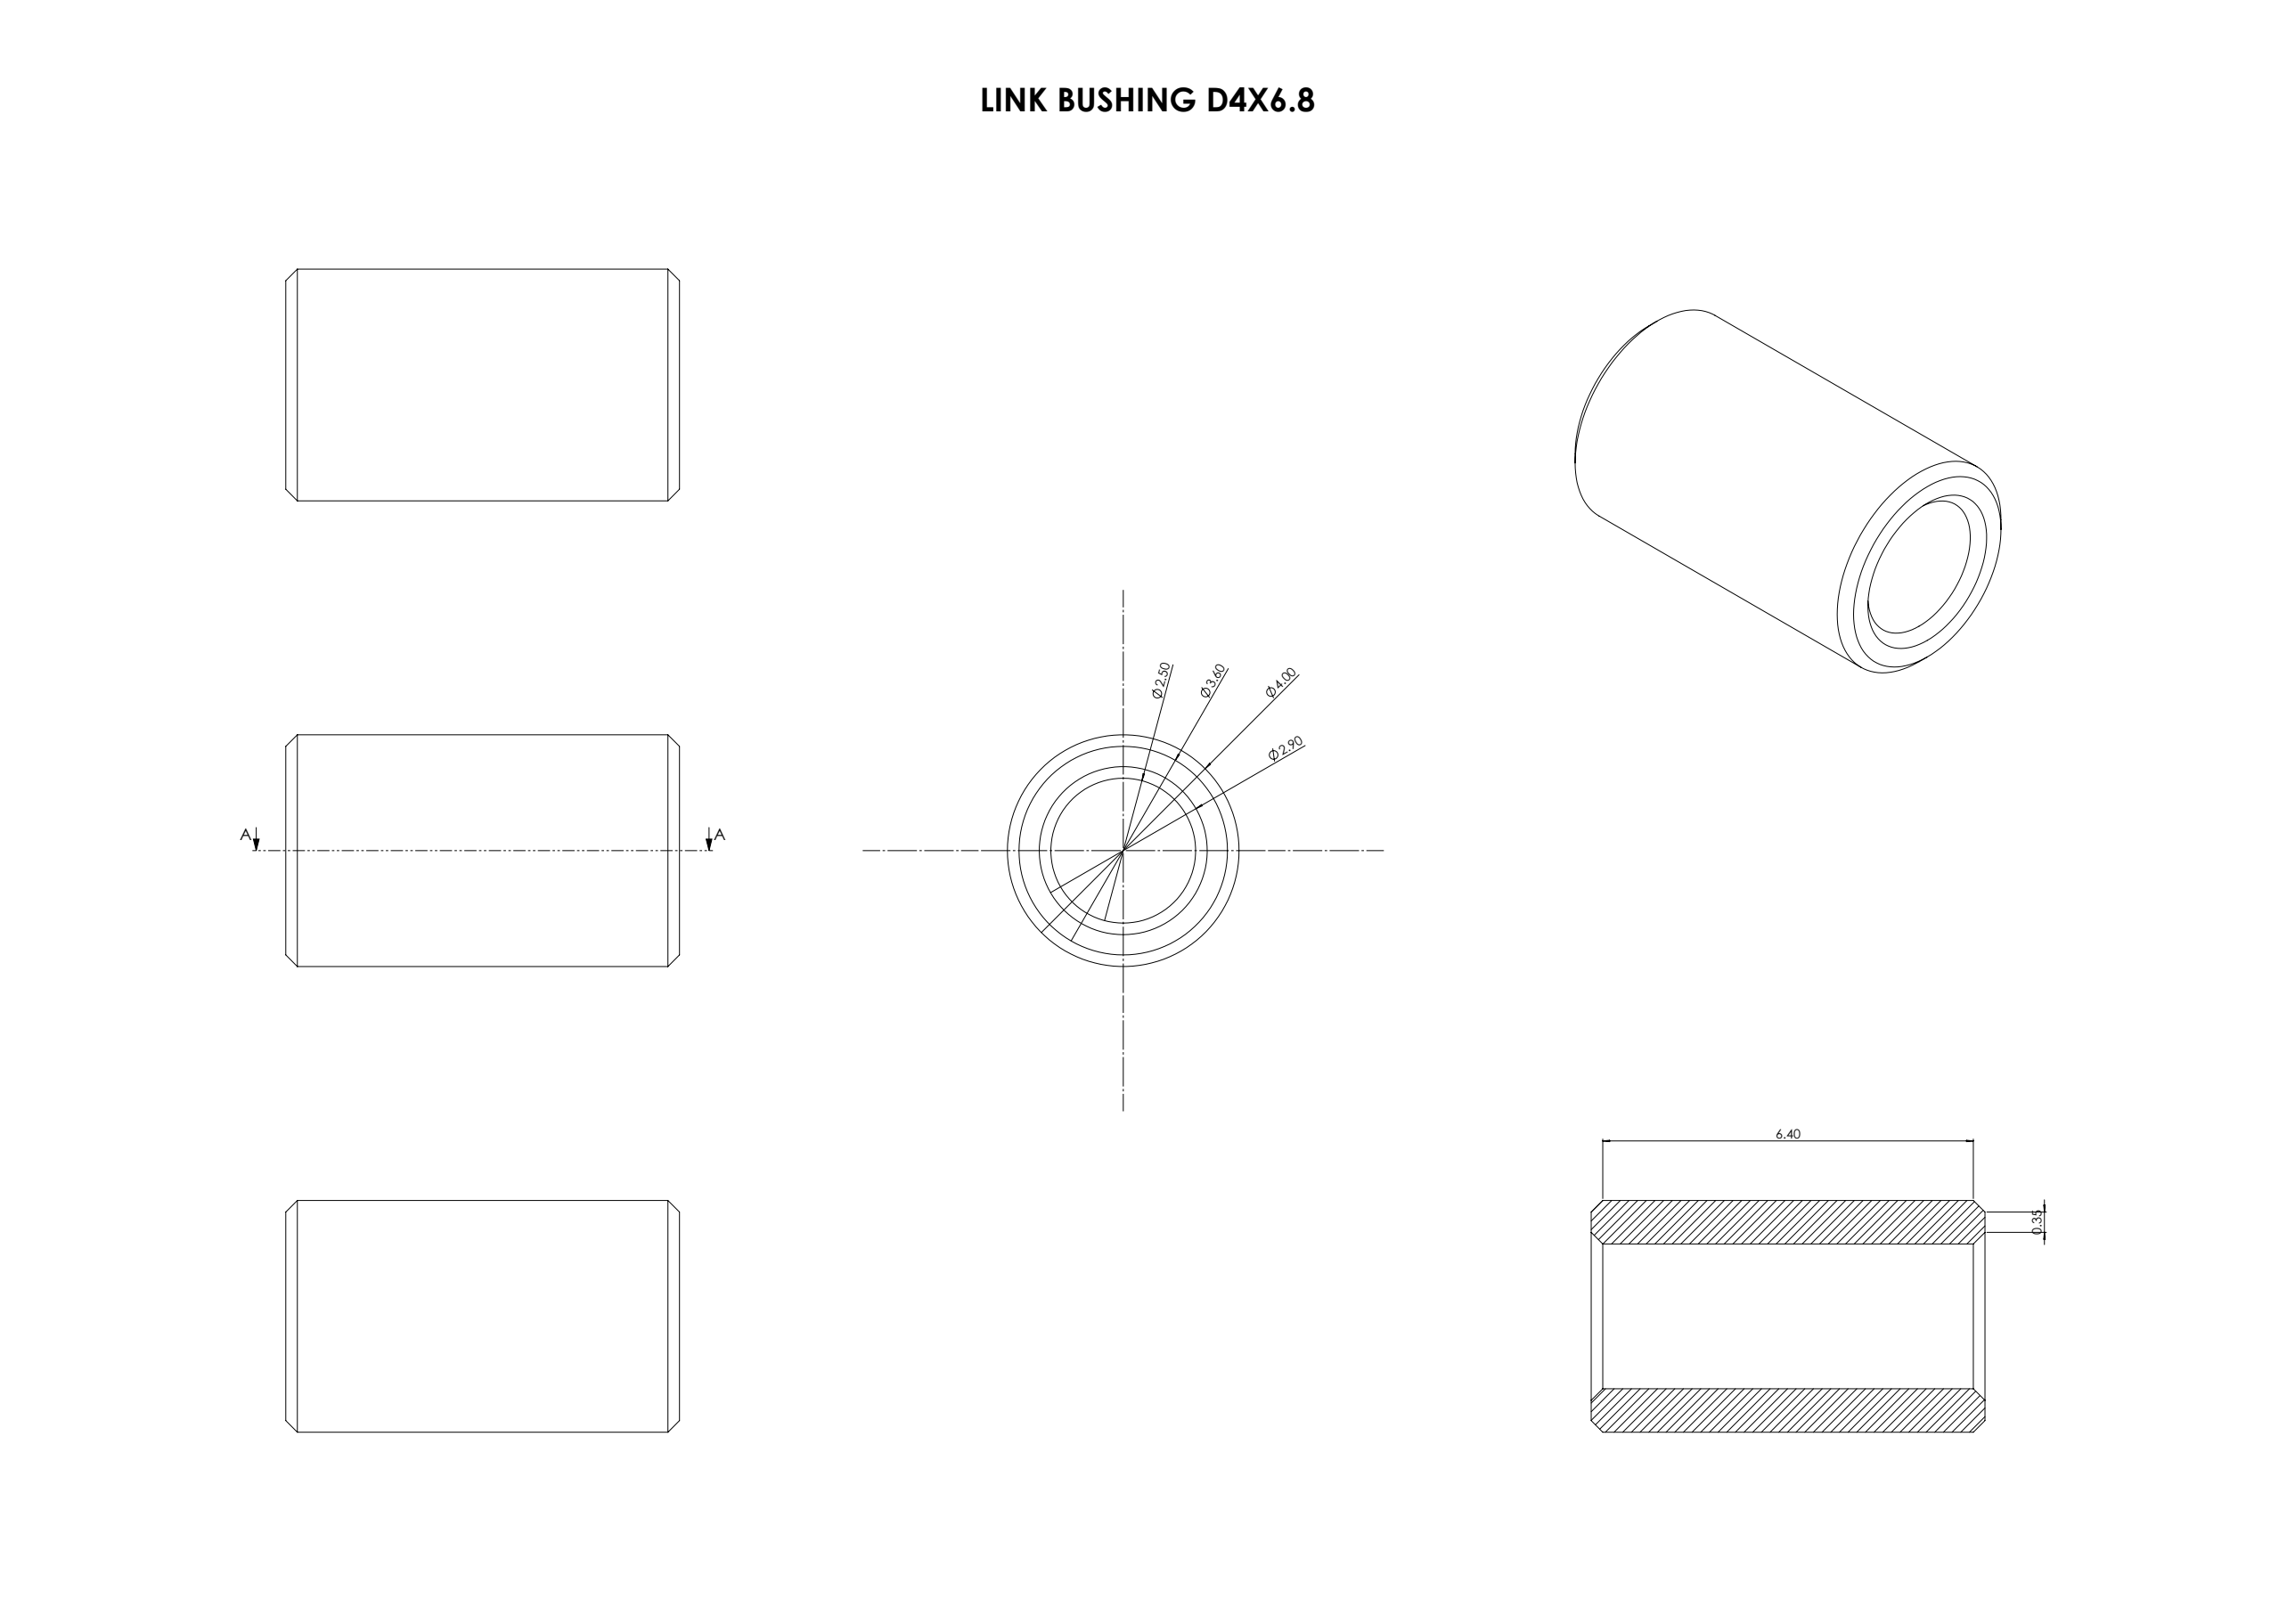
ISO-10303-21;
HEADER;
/* Generated by software containing ST-Developer
 * from STEP Tools, Inc. (www.steptools.com) 
 */

FILE_DESCRIPTION(
/* description */ (''),
/* implementation_level */ '2;1');

FILE_NAME(
/* name */ '10_Link_Bushing_D4x6.8.step',
/* time_stamp */ '2026-10-25T01:35:35-07:00',
/* author */ (''),
/* organization */ (''),
/* preprocessor_version */ 'ST-DEVELOPER v20.2',
/* originating_system */ 'Autodesk Translation Framework v15.15.0.0',
/* authorisation */ '');

FILE_SCHEMA (('AUTOMOTIVE_DESIGN { 1 0 10303 214 3 1 1 }'));
ENDSEC;

DATA;
#10=MECHANICAL_DESIGN_GEOMETRIC_PRESENTATION_REPRESENTATION('',(#271),#11430);
#247=SHAPE_REPRESENTATION_RELATIONSHIP('SRR','None',#11490,#259);
#259=ADVANCED_BREP_SHAPE_REPRESENTATION('',(#283),#11429);
#271=STYLED_ITEM('',(#11623),#283);
#283=MANIFOLD_SOLID_BREP('Body1',#4472);
#321=FACE_BOUND('',#1094,.T.);
#322=FACE_BOUND('',#1097,.T.);
#429=PLANE('',#5055);
#430=PLANE('',#5059);
#524=CYLINDRICAL_SURFACE('',#5052,1.25);
#525=CYLINDRICAL_SURFACE('',#5063,2.);
#786=FACE_OUTER_BOUND('',#1091,.T.);
#787=FACE_OUTER_BOUND('',#1092,.T.);
#788=FACE_OUTER_BOUND('',#1093,.T.);
#789=FACE_OUTER_BOUND('',#1095,.T.);
#790=FACE_OUTER_BOUND('',#1096,.T.);
#791=FACE_OUTER_BOUND('',#1098,.T.);
#792=FACE_OUTER_BOUND('',#1099,.T.);
#793=FACE_OUTER_BOUND('',#1100,.T.);
#1091=EDGE_LOOP('',(#4103,#4104,#4105,#4106,#4107));
#1092=EDGE_LOOP('',(#4108,#4109,#4110,#4111,#4112,#4113));
#1093=EDGE_LOOP('',(#4114));
#1094=EDGE_LOOP('',(#4115));
#1095=EDGE_LOOP('',(#4116,#4117,#4118,#4119,#4120));
#1096=EDGE_LOOP('',(#4121));
#1097=EDGE_LOOP('',(#4122));
#1098=EDGE_LOOP('',(#4123,#4124,#4125,#4126));
#1099=EDGE_LOOP('',(#4127,#4128,#4129,#4130));
#1100=EDGE_LOOP('',(#4131,#4132,#4133,#4134));
#1385=LINE('',#11356,#1675);
#1386=LINE('',#11365,#1676);
#1387=LINE('',#11371,#1677);
#1388=LINE('',#11379,#1678);
#1389=LINE('',#11383,#1679);
#1390=LINE('',#11385,#1680);
#1675=VECTOR('',#6255,1.35);
#1676=VECTOR('',#6266,1.25);
#1677=VECTOR('',#6273,1.35);
#1678=VECTOR('',#6284,1.9);
#1679=VECTOR('',#6289,2.);
#1680=VECTOR('',#6292,1.9);
#1856=CIRCLE('',#5049,1.45);
#1857=CIRCLE('',#5050,1.25);
#1858=CIRCLE('',#5051,1.25);
#1859=CIRCLE('',#5053,1.25);
#1860=CIRCLE('',#5054,1.25);
#1861=CIRCLE('',#5056,1.8);
#1862=CIRCLE('',#5058,1.45);
#1863=CIRCLE('',#5060,1.8);
#1864=CIRCLE('',#5062,2.);
#1865=CIRCLE('',#5064,2.);
#2250=VERTEX_POINT('',#11353);
#2251=VERTEX_POINT('',#11355);
#2252=VERTEX_POINT('',#11357);
#2253=VERTEX_POINT('',#11361);
#2254=VERTEX_POINT('',#11362);
#2255=VERTEX_POINT('',#11367);
#2256=VERTEX_POINT('',#11370);
#2257=VERTEX_POINT('',#11374);
#2258=VERTEX_POINT('',#11377);
#2259=VERTEX_POINT('',#11381);
#2869=EDGE_CURVE('',#2250,#2250,#1856,.T.);
#2870=EDGE_CURVE('',#2250,#2251,#1385,.T.);
#2871=EDGE_CURVE('',#2251,#2252,#1857,.T.);
#2872=EDGE_CURVE('',#2252,#2251,#1858,.T.);
#2873=EDGE_CURVE('',#2253,#2254,#1859,.T.);
#2874=EDGE_CURVE('',#2254,#2253,#1860,.T.);
#2875=EDGE_CURVE('',#2254,#2252,#1386,.T.);
#2876=EDGE_CURVE('',#2255,#2255,#1861,.T.);
#2877=EDGE_CURVE('',#2253,#2256,#1387,.T.);
#2878=EDGE_CURVE('',#2256,#2256,#1862,.T.);
#2879=EDGE_CURVE('',#2257,#2257,#1863,.T.);
#2880=EDGE_CURVE('',#2258,#2258,#1864,.T.);
#2881=EDGE_CURVE('',#2258,#2255,#1388,.T.);
#2882=EDGE_CURVE('',#2259,#2259,#1865,.T.);
#2883=EDGE_CURVE('',#2259,#2258,#1389,.T.);
#2884=EDGE_CURVE('',#2257,#2259,#1390,.T.);
#4103=ORIENTED_EDGE('',*,*,#2869,.T.);
#4104=ORIENTED_EDGE('',*,*,#2870,.T.);
#4105=ORIENTED_EDGE('',*,*,#2871,.T.);
#4106=ORIENTED_EDGE('',*,*,#2872,.T.);
#4107=ORIENTED_EDGE('',*,*,#2870,.F.);
#4108=ORIENTED_EDGE('',*,*,#2873,.F.);
#4109=ORIENTED_EDGE('',*,*,#2874,.F.);
#4110=ORIENTED_EDGE('',*,*,#2875,.T.);
#4111=ORIENTED_EDGE('',*,*,#2871,.F.);
#4112=ORIENTED_EDGE('',*,*,#2872,.F.);
#4113=ORIENTED_EDGE('',*,*,#2875,.F.);
#4114=ORIENTED_EDGE('',*,*,#2876,.F.);
#4115=ORIENTED_EDGE('',*,*,#2869,.F.);
#4116=ORIENTED_EDGE('',*,*,#2873,.T.);
#4117=ORIENTED_EDGE('',*,*,#2874,.T.);
#4118=ORIENTED_EDGE('',*,*,#2877,.T.);
#4119=ORIENTED_EDGE('',*,*,#2878,.T.);
#4120=ORIENTED_EDGE('',*,*,#2877,.F.);
#4121=ORIENTED_EDGE('',*,*,#2879,.T.);
#4122=ORIENTED_EDGE('',*,*,#2878,.F.);
#4123=ORIENTED_EDGE('',*,*,#2880,.F.);
#4124=ORIENTED_EDGE('',*,*,#2881,.T.);
#4125=ORIENTED_EDGE('',*,*,#2876,.T.);
#4126=ORIENTED_EDGE('',*,*,#2881,.F.);
#4127=ORIENTED_EDGE('',*,*,#2882,.F.);
#4128=ORIENTED_EDGE('',*,*,#2883,.T.);
#4129=ORIENTED_EDGE('',*,*,#2880,.T.);
#4130=ORIENTED_EDGE('',*,*,#2883,.F.);
#4131=ORIENTED_EDGE('',*,*,#2879,.F.);
#4132=ORIENTED_EDGE('',*,*,#2884,.T.);
#4133=ORIENTED_EDGE('',*,*,#2882,.T.);
#4134=ORIENTED_EDGE('',*,*,#2884,.F.);
#4189=CONICAL_SURFACE('',#5048,1.35,0.785398163397448);
#4190=CONICAL_SURFACE('',#5057,1.35,0.785398163397448);
#4191=CONICAL_SURFACE('',#5061,1.9,0.785398163397449);
#4192=CONICAL_SURFACE('',#5065,1.9,0.785398163397448);
#4453=ADVANCED_FACE('',(#786),#4189,.F.);
#4454=ADVANCED_FACE('',(#787),#524,.F.);
#4455=ADVANCED_FACE('',(#788,#321),#429,.T.);
#4456=ADVANCED_FACE('',(#789),#4190,.F.);
#4457=ADVANCED_FACE('',(#790,#322),#430,.T.);
#4458=ADVANCED_FACE('',(#791),#4191,.T.);
#4459=ADVANCED_FACE('',(#792),#525,.T.);
#4460=ADVANCED_FACE('',(#793),#4192,.T.);
#4472=CLOSED_SHELL('',(#4453,#4454,#4455,#4456,#4457,#4458,#4459,#4460));
#5047=AXIS2_PLACEMENT_3D('',#11351,#6249,#6250);
#5048=AXIS2_PLACEMENT_3D('',#11352,#6251,#6252);
#5049=AXIS2_PLACEMENT_3D('',#11354,#6253,#6254);
#5050=AXIS2_PLACEMENT_3D('',#11358,#6256,#6257);
#5051=AXIS2_PLACEMENT_3D('',#11359,#6258,#6259);
#5052=AXIS2_PLACEMENT_3D('',#11360,#6260,#6261);
#5053=AXIS2_PLACEMENT_3D('',#11363,#6262,#6263);
#5054=AXIS2_PLACEMENT_3D('',#11364,#6264,#6265);
#5055=AXIS2_PLACEMENT_3D('',#11366,#6267,#6268);
#5056=AXIS2_PLACEMENT_3D('',#11368,#6269,#6270);
#5057=AXIS2_PLACEMENT_3D('',#11369,#6271,#6272);
#5058=AXIS2_PLACEMENT_3D('',#11372,#6274,#6275);
#5059=AXIS2_PLACEMENT_3D('',#11373,#6276,#6277);
#5060=AXIS2_PLACEMENT_3D('',#11375,#6278,#6279);
#5061=AXIS2_PLACEMENT_3D('',#11376,#6280,#6281);
#5062=AXIS2_PLACEMENT_3D('',#11378,#6282,#6283);
#5063=AXIS2_PLACEMENT_3D('',#11380,#6285,#6286);
#5064=AXIS2_PLACEMENT_3D('',#11382,#6287,#6288);
#5065=AXIS2_PLACEMENT_3D('',#11384,#6290,#6291);
#6249=DIRECTION('axis',(0.,0.,1.));
#6250=DIRECTION('refdir',(1.,0.,0.));
#6251=DIRECTION('center_axis',(-1.,0.,0.));
#6252=DIRECTION('ref_axis',(0.,-1.,0.));
#6253=DIRECTION('center_axis',(-1.,0.,0.));
#6254=DIRECTION('ref_axis',(0.,-1.,0.));
#6255=DIRECTION('',(0.707106781186548,-0.707106781186548,8.65956056235493E-17));
#6256=DIRECTION('center_axis',(1.,0.,0.));
#6257=DIRECTION('ref_axis',(0.,-1.,0.));
#6258=DIRECTION('center_axis',(1.,0.,0.));
#6259=DIRECTION('ref_axis',(0.,-1.,0.));
#6260=DIRECTION('center_axis',(1.,0.,0.));
#6261=DIRECTION('ref_axis',(0.,1.,0.));
#6262=DIRECTION('center_axis',(-1.,0.,0.));
#6263=DIRECTION('ref_axis',(0.,-1.,0.));
#6264=DIRECTION('center_axis',(-1.,0.,0.));
#6265=DIRECTION('ref_axis',(0.,-1.,0.));
#6266=DIRECTION('',(-1.,0.,0.));
#6267=DIRECTION('center_axis',(-1.,0.,0.));
#6268=DIRECTION('ref_axis',(0.,0.,1.));
#6269=DIRECTION('center_axis',(1.,0.,0.));
#6270=DIRECTION('ref_axis',(0.,0.,-1.));
#6271=DIRECTION('center_axis',(1.,0.,0.));
#6272=DIRECTION('ref_axis',(0.,-1.,0.));
#6273=DIRECTION('',(0.707106781186548,0.707106781186548,-8.65956056235493E-17));
#6274=DIRECTION('center_axis',(1.,0.,0.));
#6275=DIRECTION('ref_axis',(0.,-1.,0.));
#6276=DIRECTION('center_axis',(1.,0.,0.));
#6277=DIRECTION('ref_axis',(0.,0.,-1.));
#6278=DIRECTION('center_axis',(1.,0.,0.));
#6279=DIRECTION('ref_axis',(0.,0.,-1.));
#6280=DIRECTION('center_axis',(1.,0.,0.));
#6281=DIRECTION('ref_axis',(0.,1.,0.));
#6282=DIRECTION('center_axis',(1.,0.,0.));
#6283=DIRECTION('ref_axis',(0.,0.,-1.));
#6284=DIRECTION('',(-0.707106781186547,0.707106781186548,8.65956056235494E-17));
#6285=DIRECTION('center_axis',(1.,0.,0.));
#6286=DIRECTION('ref_axis',(0.,1.,0.));
#6287=DIRECTION('center_axis',(1.,0.,0.));
#6288=DIRECTION('ref_axis',(0.,0.,-1.));
#6289=DIRECTION('',(-1.,0.,0.));
#6290=DIRECTION('center_axis',(-1.,0.,0.));
#6291=DIRECTION('ref_axis',(0.,1.,0.));
#6292=DIRECTION('',(-0.707106781186547,-0.707106781186547,-8.65956056235493E-17));
#11351=CARTESIAN_POINT('',(0.,0.,0.));
#11352=CARTESIAN_POINT('Origin',(0.1,0.,0.));
#11353=CARTESIAN_POINT('',(0.,1.45,-1.77573785876366E-16));
#11354=CARTESIAN_POINT('Origin',(0.,0.,0.));
#11355=CARTESIAN_POINT('',(0.2,1.25,1.53080849893419E-16));
#11356=CARTESIAN_POINT('',(0.1,1.35,-1.65327317884893E-16));
#11357=CARTESIAN_POINT('',(0.2,-1.25,-1.53080849893419E-16));
#11358=CARTESIAN_POINT('Origin',(0.2,0.,0.));
#11359=CARTESIAN_POINT('Origin',(0.2,0.,0.));
#11360=CARTESIAN_POINT('Origin',(3.4,0.,0.));
#11361=CARTESIAN_POINT('',(6.6,1.25,-1.53080849893419E-16));
#11362=CARTESIAN_POINT('',(6.6,-1.25,-1.53080849893419E-16));
#11363=CARTESIAN_POINT('Origin',(6.6,0.,0.));
#11364=CARTESIAN_POINT('Origin',(6.6,0.,0.));
#11365=CARTESIAN_POINT('',(3.4,-1.25,-1.53080849893419E-16));
#11366=CARTESIAN_POINT('Origin',(0.,1.8,0.));
#11367=CARTESIAN_POINT('',(1.73472347597681E-17,-1.8,-2.20436423846524E-16));
#11368=CARTESIAN_POINT('Origin',(0.,0.,0.));
#11369=CARTESIAN_POINT('Origin',(6.7,0.,0.));
#11370=CARTESIAN_POINT('',(6.8,1.45,1.77573785876366E-16));
#11371=CARTESIAN_POINT('',(6.7,1.35,-1.65327317884893E-16));
#11372=CARTESIAN_POINT('Origin',(6.8,0.,0.));
#11373=CARTESIAN_POINT('Origin',(6.8,1.25,0.));
#11374=CARTESIAN_POINT('',(6.8,-1.8,-2.20436423846524E-16));
#11375=CARTESIAN_POINT('Origin',(6.8,0.,0.));
#11376=CARTESIAN_POINT('Origin',(0.1,0.,0.));
#11377=CARTESIAN_POINT('',(0.2,-2.,-2.44929359829471E-16));
#11378=CARTESIAN_POINT('Origin',(0.2,0.,0.));
#11379=CARTESIAN_POINT('',(0.1,-1.9,-2.32682891837997E-16));
#11380=CARTESIAN_POINT('Origin',(3.4,0.,0.));
#11381=CARTESIAN_POINT('',(6.6,-2.,-2.44929359829471E-16));
#11382=CARTESIAN_POINT('Origin',(6.6,0.,0.));
#11383=CARTESIAN_POINT('',(3.4,-2.,-2.44929359829471E-16));
#11384=CARTESIAN_POINT('Origin',(6.7,0.,0.));
#11385=CARTESIAN_POINT('',(6.7,-1.9,-2.32682891837997E-16));
#11415=UNCERTAINTY_MEASURE_WITH_UNIT(LENGTH_MEASURE(0.01),#11431,
'DISTANCE_ACCURACY_VALUE',
'Maximum model space distance between geometric entities at asserted c
onnectivities');
#11416=UNCERTAINTY_MEASURE_WITH_UNIT(LENGTH_MEASURE(0.01),#11431,
'DISTANCE_ACCURACY_VALUE',
'Maximum model space distance between geometric entities at asserted c
onnectivities');
#11429=(
GEOMETRIC_REPRESENTATION_CONTEXT(3)
GLOBAL_UNCERTAINTY_ASSIGNED_CONTEXT((#11415))
GLOBAL_UNIT_ASSIGNED_CONTEXT((#11431,#11433,#11434))
REPRESENTATION_CONTEXT('','3D')
);
#11430=(
GEOMETRIC_REPRESENTATION_CONTEXT(3)
GLOBAL_UNCERTAINTY_ASSIGNED_CONTEXT((#11416))
GLOBAL_UNIT_ASSIGNED_CONTEXT((#11431,#11433,#11434))
REPRESENTATION_CONTEXT('','3D')
);
#11431=(
LENGTH_UNIT()
NAMED_UNIT(*)
SI_UNIT(.MILLI.,.METRE.)
);
#11433=(
NAMED_UNIT(*)
PLANE_ANGLE_UNIT()
SI_UNIT($,.RADIAN.)
);
#11434=(
NAMED_UNIT(*)
SI_UNIT($,.STERADIAN.)
SOLID_ANGLE_UNIT()
);
#11447=SHAPE_DEFINITION_REPRESENTATION(#11460,#11490);
#11460=PRODUCT_DEFINITION_SHAPE('',$,#11504);
#11490=SHAPE_REPRESENTATION('',(#5047),#11429);
#11491=PRODUCT_DEFINITION_CONTEXT('part definition',#11532,'design');
#11504=PRODUCT_DEFINITION('2026-10-25-00-55-40-595',
'10_Link_Bushing_D4x6.8',#11517,#11491);
#11517=PRODUCT_DEFINITION_FORMATION('',$,#11546);
#11532=APPLICATION_CONTEXT(
'Core Data for Automotive Mechanical Design Process');
#11533=PRODUCT_CONTEXT('part definition',#11532,'mechanical');
#11546=PRODUCT('2026-10-25-00-55-40-595','10_Link_Bushing_D4x6.8',$,(#11533));
#11617=COLOUR_RGB('Off White',0.89,0.88,0.83);
#11618=FILL_AREA_STYLE_COLOUR('',#11617);
#11619=FILL_AREA_STYLE('',(#11618));
#11620=SURFACE_STYLE_FILL_AREA(#11619);
#11621=SURFACE_SIDE_STYLE('',(#11620));
#11622=SURFACE_STYLE_USAGE(.BOTH.,#11621);
#11623=PRESENTATION_STYLE_ASSIGNMENT((#11622));
ENDSEC;
END-ISO-10303-21;
